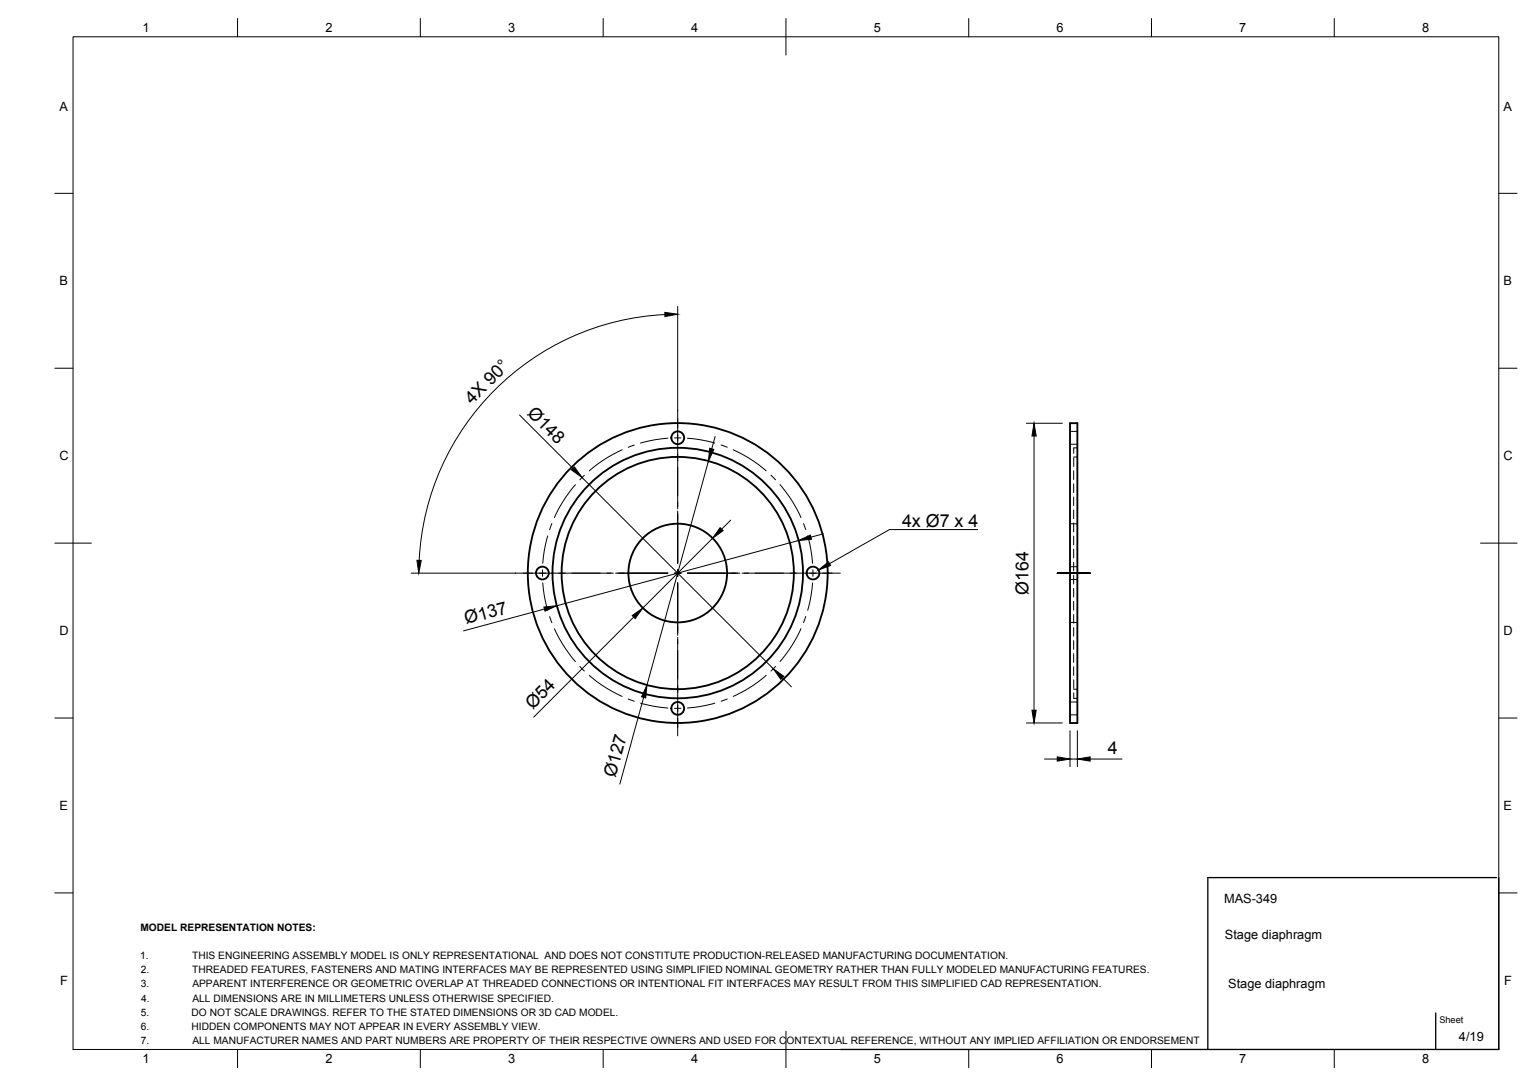
ISO-10303-21;
HEADER;
/* Generated by software containing ST-Developer
 * from STEP Tools, Inc. (www.steptools.com) 
 */

FILE_DESCRIPTION(
/* description */ ('Independent two-stage semi-open centrifugal-pump CAD. Shared impeller
s, open-machinable return casings, removable diaphragms, bronze wear/j
ournal rings, volume-preserving seal instances, retained keyed shaft, 
opposed mechanical face rings and partly threaded tie hardware. Native
 shaft rotation. Geometric topology/clearance only; flow/head/efficien
cy, pressure, cavitation, balance, preload, face loading and secondary
 seal fits/bonds, material/thermal/tolerance selection and life unassi
gned. External drive, coupling, anchors and piping bolts omitted.'),
/* implementation_level */ '2;1');

FILE_NAME(
/* name */ 'Stage diaphragm.step',
/* time_stamp */ '2026-11-08T18:06:32-08:00',
/* author */ (''),
/* organization */ (''),
/* preprocessor_version */ 'ST-DEVELOPER v20.2',
/* originating_system */ 'Autodesk Translation Framework v15.17.0.0',
/* authorisation */ '');

FILE_SCHEMA (('AUTOMOTIVE_DESIGN { 1 0 10303 214 3 1 1 }'));
ENDSEC;

DATA;
#10=MECHANICAL_DESIGN_GEOMETRIC_PRESENTATION_REPRESENTATION('',(#394),#16687);
#356=SHAPE_REPRESENTATION_RELATIONSHIP('SRR','None',#16765,#375);
#375=ADVANCED_BREP_SHAPE_REPRESENTATION('',(#413),#16669);
#394=STYLED_ITEM('',(#16869),#413);
#413=MANIFOLD_SOLID_BREP('Body1',#6113);
#454=FACE_BOUND('',#1113,.T.);
#455=FACE_BOUND('',#1115,.T.);
#456=FACE_BOUND('',#1123,.T.);
#457=FACE_BOUND('',#1124,.T.);
#458=FACE_BOUND('',#1125,.T.);
#459=FACE_BOUND('',#1126,.T.);
#460=FACE_BOUND('',#1127,.T.);
#461=FACE_BOUND('',#1129,.T.);
#462=FACE_BOUND('',#1130,.T.);
#463=FACE_BOUND('',#1131,.T.);
#464=FACE_BOUND('',#1132,.T.);
#465=FACE_BOUND('',#1133,.T.);
#583=PLANE('',#6458);
#584=PLANE('',#6459);
#585=PLANE('',#6478);
#586=PLANE('',#6479);
#740=FACE_OUTER_BOUND('',#1110,.T.);
#741=FACE_OUTER_BOUND('',#1111,.T.);
#742=FACE_OUTER_BOUND('',#1112,.T.);
#743=FACE_OUTER_BOUND('',#1114,.T.);
#744=FACE_OUTER_BOUND('',#1116,.T.);
#745=FACE_OUTER_BOUND('',#1117,.T.);
#746=FACE_OUTER_BOUND('',#1118,.T.);
#747=FACE_OUTER_BOUND('',#1119,.T.);
#748=FACE_OUTER_BOUND('',#1120,.T.);
#749=FACE_OUTER_BOUND('',#1121,.T.);
#750=FACE_OUTER_BOUND('',#1122,.T.);
#751=FACE_OUTER_BOUND('',#1128,.T.);
#1110=EDGE_LOOP('',(#4161,#4162,#4163,#4164));
#1111=EDGE_LOOP('',(#4165,#4166,#4167,#4168));
#1112=EDGE_LOOP('',(#4169));
#1113=EDGE_LOOP('',(#4170));
#1114=EDGE_LOOP('',(#4171));
#1115=EDGE_LOOP('',(#4172));
#1116=EDGE_LOOP('',(#4173,#4174,#4175,#4176));
#1117=EDGE_LOOP('',(#4177,#4178,#4179,#4180));
#1118=EDGE_LOOP('',(#4181,#4182,#4183,#4184));
#1119=EDGE_LOOP('',(#4185,#4186,#4187,#4188));
#1120=EDGE_LOOP('',(#4189,#4190,#4191,#4192));
#1121=EDGE_LOOP('',(#4193,#4194,#4195,#4196));
#1122=EDGE_LOOP('',(#4197));
#1123=EDGE_LOOP('',(#4198));
#1124=EDGE_LOOP('',(#4199));
#1125=EDGE_LOOP('',(#4200));
#1126=EDGE_LOOP('',(#4201));
#1127=EDGE_LOOP('',(#4202));
#1128=EDGE_LOOP('',(#4203));
#1129=EDGE_LOOP('',(#4204));
#1130=EDGE_LOOP('',(#4205));
#1131=EDGE_LOOP('',(#4206));
#1132=EDGE_LOOP('',(#4207));
#1133=EDGE_LOOP('',(#4208));
#1583=LINE('',#8937,#1952);
#1584=LINE('',#8943,#1953);
#1585=LINE('',#8953,#1954);
#1586=LINE('',#8959,#1955);
#1587=LINE('',#8965,#1956);
#1588=LINE('',#8971,#1957);
#1589=LINE('',#8975,#1958);
#1590=LINE('',#8981,#1959);
#1952=VECTOR('',#7295,6.35);
#1953=VECTOR('',#7302,6.85);
#1954=VECTOR('',#7315,0.35);
#1955=VECTOR('',#7322,0.35);
#1956=VECTOR('',#7329,0.35);
#1957=VECTOR('',#7336,0.35);
#1958=VECTOR('',#7341,2.7);
#1959=VECTOR('',#7348,8.2);
#2294=CIRCLE('',#6453,6.35);
#2295=CIRCLE('',#6454,6.35);
#2296=CIRCLE('',#6456,6.85);
#2297=CIRCLE('',#6457,6.85);
#2298=CIRCLE('',#6460,2.7);
#2299=CIRCLE('',#6462,0.35);
#2300=CIRCLE('',#6463,0.35);
#2301=CIRCLE('',#6465,0.35);
#2302=CIRCLE('',#6466,0.35);
#2303=CIRCLE('',#6468,0.35);
#2304=CIRCLE('',#6469,0.35);
#2305=CIRCLE('',#6471,0.35);
#2306=CIRCLE('',#6472,0.35);
#2307=CIRCLE('',#6474,2.7);
#2308=CIRCLE('',#6476,8.2);
#2309=CIRCLE('',#6477,8.2);
#2589=VERTEX_POINT('',#8934);
#2590=VERTEX_POINT('',#8936);
#2591=VERTEX_POINT('',#8940);
#2592=VERTEX_POINT('',#8942);
#2593=VERTEX_POINT('',#8947);
#2594=VERTEX_POINT('',#8950);
#2595=VERTEX_POINT('',#8952);
#2596=VERTEX_POINT('',#8956);
#2597=VERTEX_POINT('',#8958);
#2598=VERTEX_POINT('',#8962);
#2599=VERTEX_POINT('',#8964);
#2600=VERTEX_POINT('',#8968);
#2601=VERTEX_POINT('',#8970);
#2602=VERTEX_POINT('',#8974);
#2603=VERTEX_POINT('',#8978);
#2604=VERTEX_POINT('',#8980);
#3190=EDGE_CURVE('',#2589,#2589,#2294,.T.);
#3191=EDGE_CURVE('',#2589,#2590,#1583,.T.);
#3192=EDGE_CURVE('',#2590,#2590,#2295,.T.);
#3193=EDGE_CURVE('',#2591,#2591,#2296,.T.);
#3194=EDGE_CURVE('',#2591,#2592,#1584,.T.);
#3195=EDGE_CURVE('',#2592,#2592,#2297,.T.);
#3196=EDGE_CURVE('',#2593,#2593,#2298,.T.);
#3197=EDGE_CURVE('',#2594,#2594,#2299,.T.);
#3198=EDGE_CURVE('',#2594,#2595,#1585,.T.);
#3199=EDGE_CURVE('',#2595,#2595,#2300,.T.);
#3200=EDGE_CURVE('',#2596,#2596,#2301,.T.);
#3201=EDGE_CURVE('',#2596,#2597,#1586,.T.);
#3202=EDGE_CURVE('',#2597,#2597,#2302,.T.);
#3203=EDGE_CURVE('',#2598,#2598,#2303,.T.);
#3204=EDGE_CURVE('',#2598,#2599,#1587,.T.);
#3205=EDGE_CURVE('',#2599,#2599,#2304,.T.);
#3206=EDGE_CURVE('',#2600,#2600,#2305,.T.);
#3207=EDGE_CURVE('',#2600,#2601,#1588,.T.);
#3208=EDGE_CURVE('',#2601,#2601,#2306,.T.);
#3209=EDGE_CURVE('',#2593,#2602,#1589,.T.);
#3210=EDGE_CURVE('',#2602,#2602,#2307,.T.);
#3211=EDGE_CURVE('',#2603,#2603,#2308,.T.);
#3212=EDGE_CURVE('',#2603,#2604,#1590,.T.);
#3213=EDGE_CURVE('',#2604,#2604,#2309,.T.);
#4161=ORIENTED_EDGE('',*,*,#3190,.F.);
#4162=ORIENTED_EDGE('',*,*,#3191,.T.);
#4163=ORIENTED_EDGE('',*,*,#3192,.T.);
#4164=ORIENTED_EDGE('',*,*,#3191,.F.);
#4165=ORIENTED_EDGE('',*,*,#3193,.F.);
#4166=ORIENTED_EDGE('',*,*,#3194,.T.);
#4167=ORIENTED_EDGE('',*,*,#3195,.T.);
#4168=ORIENTED_EDGE('',*,*,#3194,.F.);
#4169=ORIENTED_EDGE('',*,*,#3195,.F.);
#4170=ORIENTED_EDGE('',*,*,#3192,.F.);
#4171=ORIENTED_EDGE('',*,*,#3190,.T.);
#4172=ORIENTED_EDGE('',*,*,#3196,.T.);
#4173=ORIENTED_EDGE('',*,*,#3197,.F.);
#4174=ORIENTED_EDGE('',*,*,#3198,.T.);
#4175=ORIENTED_EDGE('',*,*,#3199,.F.);
#4176=ORIENTED_EDGE('',*,*,#3198,.F.);
#4177=ORIENTED_EDGE('',*,*,#3200,.F.);
#4178=ORIENTED_EDGE('',*,*,#3201,.T.);
#4179=ORIENTED_EDGE('',*,*,#3202,.F.);
#4180=ORIENTED_EDGE('',*,*,#3201,.F.);
#4181=ORIENTED_EDGE('',*,*,#3203,.F.);
#4182=ORIENTED_EDGE('',*,*,#3204,.T.);
#4183=ORIENTED_EDGE('',*,*,#3205,.F.);
#4184=ORIENTED_EDGE('',*,*,#3204,.F.);
#4185=ORIENTED_EDGE('',*,*,#3206,.F.);
#4186=ORIENTED_EDGE('',*,*,#3207,.T.);
#4187=ORIENTED_EDGE('',*,*,#3208,.F.);
#4188=ORIENTED_EDGE('',*,*,#3207,.F.);
#4189=ORIENTED_EDGE('',*,*,#3196,.F.);
#4190=ORIENTED_EDGE('',*,*,#3209,.T.);
#4191=ORIENTED_EDGE('',*,*,#3210,.T.);
#4192=ORIENTED_EDGE('',*,*,#3209,.F.);
#4193=ORIENTED_EDGE('',*,*,#3211,.F.);
#4194=ORIENTED_EDGE('',*,*,#3212,.T.);
#4195=ORIENTED_EDGE('',*,*,#3213,.T.);
#4196=ORIENTED_EDGE('',*,*,#3212,.F.);
#4197=ORIENTED_EDGE('',*,*,#3211,.T.);
#4198=ORIENTED_EDGE('',*,*,#3197,.T.);
#4199=ORIENTED_EDGE('',*,*,#3200,.T.);
#4200=ORIENTED_EDGE('',*,*,#3203,.T.);
#4201=ORIENTED_EDGE('',*,*,#3206,.T.);
#4202=ORIENTED_EDGE('',*,*,#3193,.T.);
#4203=ORIENTED_EDGE('',*,*,#3213,.F.);
#4204=ORIENTED_EDGE('',*,*,#3210,.F.);
#4205=ORIENTED_EDGE('',*,*,#3208,.T.);
#4206=ORIENTED_EDGE('',*,*,#3205,.T.);
#4207=ORIENTED_EDGE('',*,*,#3202,.T.);
#4208=ORIENTED_EDGE('',*,*,#3199,.T.);
#5587=CYLINDRICAL_SURFACE('',#6452,6.35);
#5588=CYLINDRICAL_SURFACE('',#6455,6.85);
#5589=CYLINDRICAL_SURFACE('',#6461,0.35);
#5590=CYLINDRICAL_SURFACE('',#6464,0.35);
#5591=CYLINDRICAL_SURFACE('',#6467,0.35);
#5592=CYLINDRICAL_SURFACE('',#6470,0.35);
#5593=CYLINDRICAL_SURFACE('',#6473,2.7);
#5594=CYLINDRICAL_SURFACE('',#6475,8.2);
#5819=ADVANCED_FACE('',(#740),#5587,.T.);
#5820=ADVANCED_FACE('',(#741),#5588,.F.);
#5821=ADVANCED_FACE('',(#742,#454),#583,.T.);
#5822=ADVANCED_FACE('',(#743,#455),#584,.T.);
#5823=ADVANCED_FACE('',(#744),#5589,.F.);
#5824=ADVANCED_FACE('',(#745),#5590,.F.);
#5825=ADVANCED_FACE('',(#746),#5591,.F.);
#5826=ADVANCED_FACE('',(#747),#5592,.F.);
#5827=ADVANCED_FACE('',(#748),#5593,.F.);
#5828=ADVANCED_FACE('',(#749),#5594,.T.);
#5829=ADVANCED_FACE('',(#750,#456,#457,#458,#459,#460),#585,.T.);
#5830=ADVANCED_FACE('',(#751,#461,#462,#463,#464,#465),#586,.F.);
#6113=CLOSED_SHELL('',(#5819,#5820,#5821,#5822,#5823,#5824,#5825,#5826,
#5827,#5828,#5829,#5830));
#6451=AXIS2_PLACEMENT_3D('',#8932,#7289,#7290);
#6452=AXIS2_PLACEMENT_3D('',#8933,#7291,#7292);
#6453=AXIS2_PLACEMENT_3D('',#8935,#7293,#7294);
#6454=AXIS2_PLACEMENT_3D('',#8938,#7296,#7297);
#6455=AXIS2_PLACEMENT_3D('',#8939,#7298,#7299);
#6456=AXIS2_PLACEMENT_3D('',#8941,#7300,#7301);
#6457=AXIS2_PLACEMENT_3D('',#8944,#7303,#7304);
#6458=AXIS2_PLACEMENT_3D('',#8945,#7305,#7306);
#6459=AXIS2_PLACEMENT_3D('',#8946,#7307,#7308);
#6460=AXIS2_PLACEMENT_3D('',#8948,#7309,#7310);
#6461=AXIS2_PLACEMENT_3D('',#8949,#7311,#7312);
#6462=AXIS2_PLACEMENT_3D('',#8951,#7313,#7314);
#6463=AXIS2_PLACEMENT_3D('',#8954,#7316,#7317);
#6464=AXIS2_PLACEMENT_3D('',#8955,#7318,#7319);
#6465=AXIS2_PLACEMENT_3D('',#8957,#7320,#7321);
#6466=AXIS2_PLACEMENT_3D('',#8960,#7323,#7324);
#6467=AXIS2_PLACEMENT_3D('',#8961,#7325,#7326);
#6468=AXIS2_PLACEMENT_3D('',#8963,#7327,#7328);
#6469=AXIS2_PLACEMENT_3D('',#8966,#7330,#7331);
#6470=AXIS2_PLACEMENT_3D('',#8967,#7332,#7333);
#6471=AXIS2_PLACEMENT_3D('',#8969,#7334,#7335);
#6472=AXIS2_PLACEMENT_3D('',#8972,#7337,#7338);
#6473=AXIS2_PLACEMENT_3D('',#8973,#7339,#7340);
#6474=AXIS2_PLACEMENT_3D('',#8976,#7342,#7343);
#6475=AXIS2_PLACEMENT_3D('',#8977,#7344,#7345);
#6476=AXIS2_PLACEMENT_3D('',#8979,#7346,#7347);
#6477=AXIS2_PLACEMENT_3D('',#8982,#7349,#7350);
#6478=AXIS2_PLACEMENT_3D('',#8983,#7351,#7352);
#6479=AXIS2_PLACEMENT_3D('',#8984,#7353,#7354);
#7289=DIRECTION('axis',(0.,0.,1.));
#7290=DIRECTION('refdir',(1.,0.,0.));
#7291=DIRECTION('center_axis',(0.,0.,-1.));
#7292=DIRECTION('ref_axis',(1.,0.,0.));
#7293=DIRECTION('center_axis',(0.,0.,1.));
#7294=DIRECTION('ref_axis',(1.,0.,0.));
#7295=DIRECTION('',(0.,0.,-1.));
#7296=DIRECTION('center_axis',(0.,0.,1.));
#7297=DIRECTION('ref_axis',(1.,0.,0.));
#7298=DIRECTION('center_axis',(0.,0.,-1.));
#7299=DIRECTION('ref_axis',(1.,0.,0.));
#7300=DIRECTION('center_axis',(0.,0.,-1.));
#7301=DIRECTION('ref_axis',(1.,0.,0.));
#7302=DIRECTION('',(0.,0.,-1.));
#7303=DIRECTION('center_axis',(0.,0.,-1.));
#7304=DIRECTION('ref_axis',(1.,0.,0.));
#7305=DIRECTION('center_axis',(0.,0.,1.));
#7306=DIRECTION('ref_axis',(1.,0.,0.));
#7307=DIRECTION('center_axis',(0.,0.,1.));
#7308=DIRECTION('ref_axis',(1.,0.,0.));
#7309=DIRECTION('center_axis',(0.,0.,-1.));
#7310=DIRECTION('ref_axis',(1.,0.,0.));
#7311=DIRECTION('center_axis',(0.,0.,-1.));
#7312=DIRECTION('ref_axis',(1.,0.,0.));
#7313=DIRECTION('center_axis',(0.,0.,-1.));
#7314=DIRECTION('ref_axis',(1.,0.,0.));
#7315=DIRECTION('',(0.,0.,-1.));
#7316=DIRECTION('center_axis',(0.,0.,1.));
#7317=DIRECTION('ref_axis',(1.,0.,0.));
#7318=DIRECTION('center_axis',(0.,0.,-1.));
#7319=DIRECTION('ref_axis',(1.,0.,0.));
#7320=DIRECTION('center_axis',(0.,0.,-1.));
#7321=DIRECTION('ref_axis',(1.,0.,0.));
#7322=DIRECTION('',(0.,0.,-1.));
#7323=DIRECTION('center_axis',(0.,0.,1.));
#7324=DIRECTION('ref_axis',(1.,0.,0.));
#7325=DIRECTION('center_axis',(0.,0.,-1.));
#7326=DIRECTION('ref_axis',(1.,0.,0.));
#7327=DIRECTION('center_axis',(0.,0.,-1.));
#7328=DIRECTION('ref_axis',(1.,0.,0.));
#7329=DIRECTION('',(0.,0.,-1.));
#7330=DIRECTION('center_axis',(0.,0.,1.));
#7331=DIRECTION('ref_axis',(1.,0.,0.));
#7332=DIRECTION('center_axis',(0.,0.,-1.));
#7333=DIRECTION('ref_axis',(1.,0.,0.));
#7334=DIRECTION('center_axis',(0.,0.,-1.));
#7335=DIRECTION('ref_axis',(1.,0.,0.));
#7336=DIRECTION('',(0.,0.,-1.));
#7337=DIRECTION('center_axis',(0.,0.,1.));
#7338=DIRECTION('ref_axis',(1.,0.,0.));
#7339=DIRECTION('center_axis',(0.,0.,1.));
#7340=DIRECTION('ref_axis',(1.,0.,0.));
#7341=DIRECTION('',(0.,0.,-1.));
#7342=DIRECTION('center_axis',(0.,0.,-1.));
#7343=DIRECTION('ref_axis',(1.,0.,0.));
#7344=DIRECTION('center_axis',(0.,0.,1.));
#7345=DIRECTION('ref_axis',(1.,0.,0.));
#7346=DIRECTION('center_axis',(0.,0.,1.));
#7347=DIRECTION('ref_axis',(1.,0.,0.));
#7348=DIRECTION('',(0.,0.,-1.));
#7349=DIRECTION('center_axis',(0.,0.,1.));
#7350=DIRECTION('ref_axis',(1.,0.,0.));
#7351=DIRECTION('center_axis',(0.,0.,1.));
#7352=DIRECTION('ref_axis',(1.,0.,0.));
#7353=DIRECTION('center_axis',(0.,0.,1.));
#7354=DIRECTION('ref_axis',(1.,0.,0.));
#8932=CARTESIAN_POINT('',(0.,0.,0.));
#8933=CARTESIAN_POINT('Origin',(0.,0.,4.2));
#8934=CARTESIAN_POINT('',(-6.35,-7.77650717458569E-16,4.2));
#8935=CARTESIAN_POINT('Origin',(0.,0.,4.2));
#8936=CARTESIAN_POINT('',(-6.35,-7.77650717458569E-16,4.));
#8937=CARTESIAN_POINT('',(-6.35,7.77650717458569E-16,4.2));
#8938=CARTESIAN_POINT('Origin',(0.,0.,4.));
#8939=CARTESIAN_POINT('Origin',(0.,0.,4.2));
#8940=CARTESIAN_POINT('',(-6.85,-8.38883057415937E-16,4.2));
#8941=CARTESIAN_POINT('Origin',(0.,0.,4.2));
#8942=CARTESIAN_POINT('',(-6.85,-8.38883057415937E-16,4.));
#8943=CARTESIAN_POINT('',(-6.85,8.38883057415937E-16,4.2));
#8944=CARTESIAN_POINT('Origin',(0.,0.,4.));
#8945=CARTESIAN_POINT('Origin',(0.,0.,4.));
#8946=CARTESIAN_POINT('Origin',(0.,0.,4.2));
#8947=CARTESIAN_POINT('',(-2.7,-3.30654635769785E-16,4.2));
#8948=CARTESIAN_POINT('Origin',(0.,0.,4.2));
#8949=CARTESIAN_POINT('Origin',(-7.4,0.,4.));
#8950=CARTESIAN_POINT('',(-7.75,4.28626379701574E-17,4.2));
#8951=CARTESIAN_POINT('Origin',(-7.4,0.,4.2));
#8952=CARTESIAN_POINT('',(-7.75,4.28626379701574E-17,3.8));
#8953=CARTESIAN_POINT('',(-7.75,4.28626379701574E-17,4.));
#8954=CARTESIAN_POINT('Origin',(-7.4,0.,3.8));
#8955=CARTESIAN_POINT('Origin',(7.4,0.,4.));
#8956=CARTESIAN_POINT('',(7.05,4.28626379701574E-17,4.2));
#8957=CARTESIAN_POINT('Origin',(7.4,0.,4.2));
#8958=CARTESIAN_POINT('',(7.05,4.28626379701574E-17,3.8));
#8959=CARTESIAN_POINT('',(7.05,4.28626379701574E-17,4.));
#8960=CARTESIAN_POINT('Origin',(7.4,0.,3.8));
#8961=CARTESIAN_POINT('Origin',(0.,7.4,4.));
#8962=CARTESIAN_POINT('',(-0.35,7.4,4.2));
#8963=CARTESIAN_POINT('Origin',(0.,7.4,4.2));
#8964=CARTESIAN_POINT('',(-0.35,7.4,3.8));
#8965=CARTESIAN_POINT('',(-0.35,7.4,4.));
#8966=CARTESIAN_POINT('Origin',(0.,7.4,3.8));
#8967=CARTESIAN_POINT('Origin',(0.,-7.4,4.));
#8968=CARTESIAN_POINT('',(-0.35,-7.4,4.2));
#8969=CARTESIAN_POINT('Origin',(0.,-7.4,4.2));
#8970=CARTESIAN_POINT('',(-0.35,-7.4,3.8));
#8971=CARTESIAN_POINT('',(-0.35,-7.4,4.));
#8972=CARTESIAN_POINT('Origin',(0.,-7.4,3.8));
#8973=CARTESIAN_POINT('Origin',(0.,0.,3.8));
#8974=CARTESIAN_POINT('',(-2.7,-3.30654635769785E-16,3.8));
#8975=CARTESIAN_POINT('',(-2.7,-3.30654635769785E-16,3.8));
#8976=CARTESIAN_POINT('Origin',(0.,0.,3.8));
#8977=CARTESIAN_POINT('Origin',(0.,0.,3.8));
#8978=CARTESIAN_POINT('',(-8.2,-1.00421037530083E-15,4.2));
#8979=CARTESIAN_POINT('Origin',(0.,0.,4.2));
#8980=CARTESIAN_POINT('',(-8.2,-1.00421037530083E-15,3.8));
#8981=CARTESIAN_POINT('',(-8.2,-1.00421037530083E-15,3.8));
#8982=CARTESIAN_POINT('Origin',(0.,0.,3.8));
#8983=CARTESIAN_POINT('Origin',(0.,0.,4.2));
#8984=CARTESIAN_POINT('Origin',(0.,0.,3.8));
#16648=UNCERTAINTY_MEASURE_WITH_UNIT(LENGTH_MEASURE(0.001),#16688,
'DISTANCE_ACCURACY_VALUE',
'Maximum model space distance between geometric entities at asserted c
onnectivities');
#16666=UNCERTAINTY_MEASURE_WITH_UNIT(LENGTH_MEASURE(0.001),#16688,
'DISTANCE_ACCURACY_VALUE',
'Maximum model space distance between geometric entities at asserted c
onnectivities');
#16669=(
GEOMETRIC_REPRESENTATION_CONTEXT(3)
GLOBAL_UNCERTAINTY_ASSIGNED_CONTEXT((#16648))
GLOBAL_UNIT_ASSIGNED_CONTEXT((#16688,#16690,#16691))
REPRESENTATION_CONTEXT('','3D')
);
#16687=(
GEOMETRIC_REPRESENTATION_CONTEXT(3)
GLOBAL_UNCERTAINTY_ASSIGNED_CONTEXT((#16666))
GLOBAL_UNIT_ASSIGNED_CONTEXT((#16688,#16690,#16691))
REPRESENTATION_CONTEXT('','3D')
);
#16688=(
LENGTH_UNIT()
NAMED_UNIT(*)
SI_UNIT(.CENTI.,.METRE.)
);
#16690=(
NAMED_UNIT(*)
PLANE_ANGLE_UNIT()
SI_UNIT($,.RADIAN.)
);
#16691=(
NAMED_UNIT(*)
SI_UNIT($,.STERADIAN.)
SOLID_ANGLE_UNIT()
);
#16694=SHAPE_DEFINITION_REPRESENTATION(#16714,#16765);
#16714=PRODUCT_DEFINITION_SHAPE('',$,#16786);
#16765=SHAPE_REPRESENTATION('',(#6451),#16669);
#16783=PRODUCT_DEFINITION_CONTEXT('part definition',#16845,'design');
#16786=PRODUCT_DEFINITION('Stage diaphragm','Stage diaphragm',#16806,#16783);
#16806=PRODUCT_DEFINITION_FORMATION('',$,#16849);
#16845=APPLICATION_CONTEXT(
'Core Data for Automotive Mechanical Design Process');
#16846=PRODUCT_CONTEXT('part definition',#16845,'mechanical');
#16849=PRODUCT('Stage diaphragm','Stage diaphragm',$,(#16846));
#16869=PRESENTATION_STYLE_ASSIGNMENT((#16884));
#16884=SURFACE_STYLE_USAGE(.BOTH.,#16899);
#16899=SURFACE_SIDE_STYLE('',(#16914));
#16914=SURFACE_STYLE_FILL_AREA(#16929);
#16929=FILL_AREA_STYLE('Sky blue',(#16944));
#16944=FILL_AREA_STYLE_COLOUR('Sky blue',#16959);
#16959=COLOUR_RGB('Sky blue',0.317647058823529,0.686274509803922,0.890196078431372);
ENDSEC;
END-ISO-10303-21;
